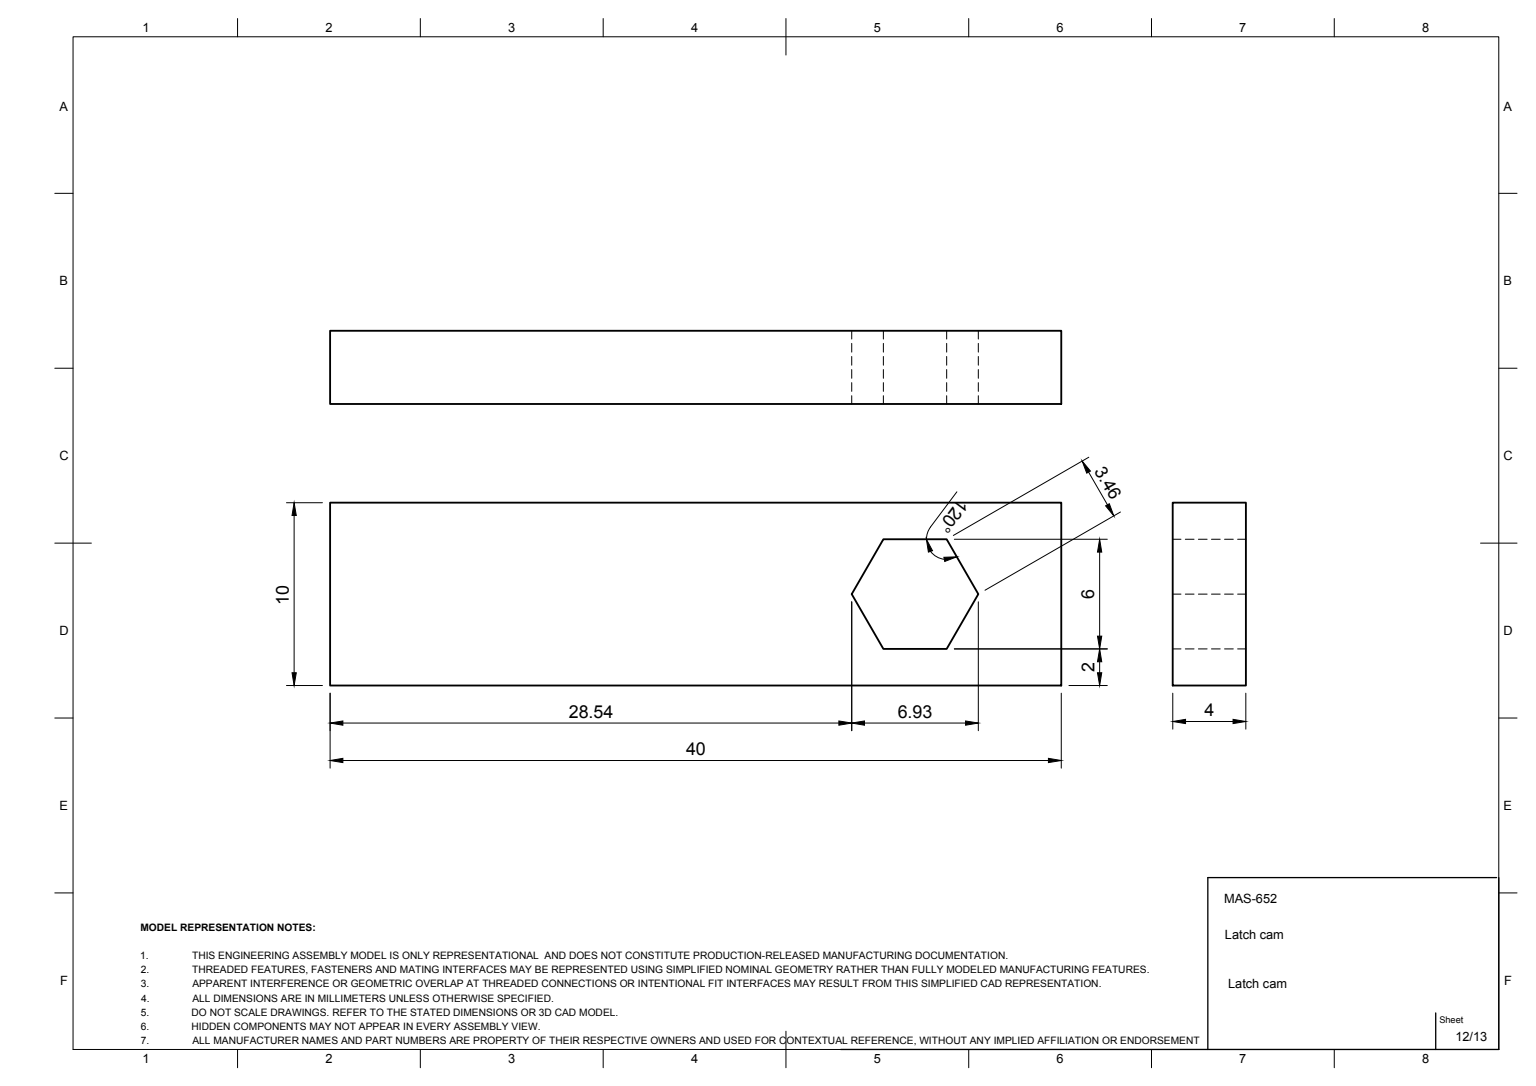
ISO-10303-21;
HEADER;
/* Generated by software containing ST-Developer
 * from STEP Tools, Inc. (www.steptools.com) 
 */

FILE_DESCRIPTION(
/* description */ ('Independent hinged machine back cover with retained hinge pins, perim
eter gasket and quarter-turn cam latch. Nominal cover 360 x 260 x 3 mm
, frame 430 x 300 x 20 mm. No guarding, structural or ingress rating a
ssigned.'),
/* implementation_level */ '2;1');

FILE_NAME(
/* name */ 'Latch cam.step',
/* time_stamp */ '2026-11-09T19:36:59-08:00',
/* author */ (''),
/* organization */ (''),
/* preprocessor_version */ 'ST-DEVELOPER v20.2',
/* originating_system */ 'Autodesk Translation Framework v15.17.0.0',
/* authorisation */ '');

FILE_SCHEMA (('AUTOMOTIVE_DESIGN { 1 0 10303 214 3 1 1 }'));
ENDSEC;

DATA;
#10=MECHANICAL_DESIGN_GEOMETRIC_PRESENTATION_REPRESENTATION('',(#202),#32627);
#166=SHAPE_REPRESENTATION_RELATIONSHIP('SRR','None',#32712,#184);
#184=ADVANCED_BREP_SHAPE_REPRESENTATION('',(#220),#32613);
#202=STYLED_ITEM('',(#32811),#220);
#220=MANIFOLD_SOLID_BREP('Body1',#8679);
#258=FACE_BOUND('',#1211,.T.);
#259=FACE_BOUND('',#1213,.T.);
#364=PLANE('',#9184);
#365=PLANE('',#9185);
#366=PLANE('',#9186);
#367=PLANE('',#9187);
#368=PLANE('',#9188);
#369=PLANE('',#9189);
#370=PLANE('',#9190);
#371=PLANE('',#9191);
#372=PLANE('',#9192);
#373=PLANE('',#9193);
#374=PLANE('',#9194);
#375=PLANE('',#9195);
#701=FACE_OUTER_BOUND('',#1200,.T.);
#702=FACE_OUTER_BOUND('',#1201,.T.);
#703=FACE_OUTER_BOUND('',#1202,.T.);
#704=FACE_OUTER_BOUND('',#1203,.T.);
#705=FACE_OUTER_BOUND('',#1204,.T.);
#706=FACE_OUTER_BOUND('',#1205,.T.);
#707=FACE_OUTER_BOUND('',#1206,.T.);
#708=FACE_OUTER_BOUND('',#1207,.T.);
#709=FACE_OUTER_BOUND('',#1208,.T.);
#710=FACE_OUTER_BOUND('',#1209,.T.);
#711=FACE_OUTER_BOUND('',#1210,.T.);
#712=FACE_OUTER_BOUND('',#1212,.T.);
#1200=EDGE_LOOP('',(#6753,#6754,#6755,#6756));
#1201=EDGE_LOOP('',(#6757,#6758,#6759,#6760));
#1202=EDGE_LOOP('',(#6761,#6762,#6763,#6764));
#1203=EDGE_LOOP('',(#6765,#6766,#6767,#6768));
#1204=EDGE_LOOP('',(#6769,#6770,#6771,#6772));
#1205=EDGE_LOOP('',(#6773,#6774,#6775,#6776));
#1206=EDGE_LOOP('',(#6777,#6778,#6779,#6780));
#1207=EDGE_LOOP('',(#6781,#6782,#6783,#6784));
#1208=EDGE_LOOP('',(#6785,#6786,#6787,#6788));
#1209=EDGE_LOOP('',(#6789,#6790,#6791,#6792));
#1210=EDGE_LOOP('',(#6793,#6794,#6795,#6796));
#1211=EDGE_LOOP('',(#6797,#6798,#6799,#6800,#6801,#6802));
#1212=EDGE_LOOP('',(#6803,#6804,#6805,#6806));
#1213=EDGE_LOOP('',(#6807,#6808,#6809,#6810,#6811,#6812));
#2446=LINE('',#24206,#2992);
#2447=LINE('',#24208,#2993);
#2448=LINE('',#24210,#2994);
#2449=LINE('',#24211,#2995);
#2450=LINE('',#24214,#2996);
#2451=LINE('',#24216,#2997);
#2452=LINE('',#24217,#2998);
#2453=LINE('',#24220,#2999);
#2454=LINE('',#24222,#3000);
#2455=LINE('',#24223,#3001);
#2456=LINE('',#24226,#3002);
#2457=LINE('',#24228,#3003);
#2458=LINE('',#24229,#3004);
#2459=LINE('',#24232,#3005);
#2460=LINE('',#24234,#3006);
#2461=LINE('',#24235,#3007);
#2462=LINE('',#24237,#3008);
#2463=LINE('',#24238,#3009);
#2464=LINE('',#24242,#3010);
#2465=LINE('',#24244,#3011);
#2466=LINE('',#24246,#3012);
#2467=LINE('',#24247,#3013);
#2468=LINE('',#24250,#3014);
#2469=LINE('',#24252,#3015);
#2470=LINE('',#24253,#3016);
#2471=LINE('',#24256,#3017);
#2472=LINE('',#24258,#3018);
#2473=LINE('',#24259,#3019);
#2474=LINE('',#24261,#3020);
#2475=LINE('',#24262,#3021);
#2992=VECTOR('',#10386,10.);
#2993=VECTOR('',#10387,10.);
#2994=VECTOR('',#10388,10.);
#2995=VECTOR('',#10389,10.);
#2996=VECTOR('',#10392,10.);
#2997=VECTOR('',#10393,10.);
#2998=VECTOR('',#10394,10.);
#2999=VECTOR('',#10397,10.);
#3000=VECTOR('',#10398,10.);
#3001=VECTOR('',#10399,10.);
#3002=VECTOR('',#10402,10.);
#3003=VECTOR('',#10403,10.);
#3004=VECTOR('',#10404,10.);
#3005=VECTOR('',#10407,10.);
#3006=VECTOR('',#10408,10.);
#3007=VECTOR('',#10409,10.);
#3008=VECTOR('',#10412,10.);
#3009=VECTOR('',#10413,10.);
#3010=VECTOR('',#10416,10.);
#3011=VECTOR('',#10417,10.);
#3012=VECTOR('',#10418,10.);
#3013=VECTOR('',#10419,10.);
#3014=VECTOR('',#10422,10.);
#3015=VECTOR('',#10423,10.);
#3016=VECTOR('',#10424,10.);
#3017=VECTOR('',#10427,10.);
#3018=VECTOR('',#10428,10.);
#3019=VECTOR('',#10429,10.);
#3020=VECTOR('',#10432,10.);
#3021=VECTOR('',#10433,10.);
#3729=VERTEX_POINT('',#24204);
#3730=VERTEX_POINT('',#24205);
#3731=VERTEX_POINT('',#24207);
#3732=VERTEX_POINT('',#24209);
#3733=VERTEX_POINT('',#24213);
#3734=VERTEX_POINT('',#24215);
#3735=VERTEX_POINT('',#24219);
#3736=VERTEX_POINT('',#24221);
#3737=VERTEX_POINT('',#24225);
#3738=VERTEX_POINT('',#24227);
#3739=VERTEX_POINT('',#24231);
#3740=VERTEX_POINT('',#24233);
#3741=VERTEX_POINT('',#24240);
#3742=VERTEX_POINT('',#24241);
#3743=VERTEX_POINT('',#24243);
#3744=VERTEX_POINT('',#24245);
#3745=VERTEX_POINT('',#24249);
#3746=VERTEX_POINT('',#24251);
#3747=VERTEX_POINT('',#24255);
#3748=VERTEX_POINT('',#24257);
#4800=EDGE_CURVE('',#3729,#3730,#2446,.T.);
#4801=EDGE_CURVE('',#3729,#3731,#2447,.T.);
#4802=EDGE_CURVE('',#3732,#3731,#2448,.T.);
#4803=EDGE_CURVE('',#3730,#3732,#2449,.T.);
#4804=EDGE_CURVE('',#3733,#3729,#2450,.T.);
#4805=EDGE_CURVE('',#3733,#3734,#2451,.T.);
#4806=EDGE_CURVE('',#3731,#3734,#2452,.T.);
#4807=EDGE_CURVE('',#3735,#3733,#2453,.T.);
#4808=EDGE_CURVE('',#3735,#3736,#2454,.T.);
#4809=EDGE_CURVE('',#3734,#3736,#2455,.T.);
#4810=EDGE_CURVE('',#3737,#3735,#2456,.T.);
#4811=EDGE_CURVE('',#3737,#3738,#2457,.T.);
#4812=EDGE_CURVE('',#3736,#3738,#2458,.T.);
#4813=EDGE_CURVE('',#3739,#3737,#2459,.T.);
#4814=EDGE_CURVE('',#3739,#3740,#2460,.T.);
#4815=EDGE_CURVE('',#3738,#3740,#2461,.T.);
#4816=EDGE_CURVE('',#3730,#3739,#2462,.T.);
#4817=EDGE_CURVE('',#3740,#3732,#2463,.T.);
#4818=EDGE_CURVE('',#3741,#3742,#2464,.T.);
#4819=EDGE_CURVE('',#3742,#3743,#2465,.T.);
#4820=EDGE_CURVE('',#3744,#3743,#2466,.T.);
#4821=EDGE_CURVE('',#3741,#3744,#2467,.T.);
#4822=EDGE_CURVE('',#3745,#3741,#2468,.T.);
#4823=EDGE_CURVE('',#3746,#3744,#2469,.T.);
#4824=EDGE_CURVE('',#3745,#3746,#2470,.T.);
#4825=EDGE_CURVE('',#3747,#3745,#2471,.T.);
#4826=EDGE_CURVE('',#3748,#3746,#2472,.T.);
#4827=EDGE_CURVE('',#3747,#3748,#2473,.T.);
#4828=EDGE_CURVE('',#3742,#3747,#2474,.T.);
#4829=EDGE_CURVE('',#3743,#3748,#2475,.T.);
#6753=ORIENTED_EDGE('',*,*,#4800,.F.);
#6754=ORIENTED_EDGE('',*,*,#4801,.T.);
#6755=ORIENTED_EDGE('',*,*,#4802,.F.);
#6756=ORIENTED_EDGE('',*,*,#4803,.F.);
#6757=ORIENTED_EDGE('',*,*,#4804,.F.);
#6758=ORIENTED_EDGE('',*,*,#4805,.T.);
#6759=ORIENTED_EDGE('',*,*,#4806,.F.);
#6760=ORIENTED_EDGE('',*,*,#4801,.F.);
#6761=ORIENTED_EDGE('',*,*,#4807,.F.);
#6762=ORIENTED_EDGE('',*,*,#4808,.T.);
#6763=ORIENTED_EDGE('',*,*,#4809,.F.);
#6764=ORIENTED_EDGE('',*,*,#4805,.F.);
#6765=ORIENTED_EDGE('',*,*,#4810,.F.);
#6766=ORIENTED_EDGE('',*,*,#4811,.T.);
#6767=ORIENTED_EDGE('',*,*,#4812,.F.);
#6768=ORIENTED_EDGE('',*,*,#4808,.F.);
#6769=ORIENTED_EDGE('',*,*,#4813,.F.);
#6770=ORIENTED_EDGE('',*,*,#4814,.T.);
#6771=ORIENTED_EDGE('',*,*,#4815,.F.);
#6772=ORIENTED_EDGE('',*,*,#4811,.F.);
#6773=ORIENTED_EDGE('',*,*,#4816,.F.);
#6774=ORIENTED_EDGE('',*,*,#4803,.T.);
#6775=ORIENTED_EDGE('',*,*,#4817,.F.);
#6776=ORIENTED_EDGE('',*,*,#4814,.F.);
#6777=ORIENTED_EDGE('',*,*,#4818,.T.);
#6778=ORIENTED_EDGE('',*,*,#4819,.T.);
#6779=ORIENTED_EDGE('',*,*,#4820,.F.);
#6780=ORIENTED_EDGE('',*,*,#4821,.F.);
#6781=ORIENTED_EDGE('',*,*,#4822,.T.);
#6782=ORIENTED_EDGE('',*,*,#4821,.T.);
#6783=ORIENTED_EDGE('',*,*,#4823,.F.);
#6784=ORIENTED_EDGE('',*,*,#4824,.F.);
#6785=ORIENTED_EDGE('',*,*,#4825,.T.);
#6786=ORIENTED_EDGE('',*,*,#4824,.T.);
#6787=ORIENTED_EDGE('',*,*,#4826,.F.);
#6788=ORIENTED_EDGE('',*,*,#4827,.F.);
#6789=ORIENTED_EDGE('',*,*,#4828,.T.);
#6790=ORIENTED_EDGE('',*,*,#4827,.T.);
#6791=ORIENTED_EDGE('',*,*,#4829,.F.);
#6792=ORIENTED_EDGE('',*,*,#4819,.F.);
#6793=ORIENTED_EDGE('',*,*,#4829,.T.);
#6794=ORIENTED_EDGE('',*,*,#4826,.T.);
#6795=ORIENTED_EDGE('',*,*,#4823,.T.);
#6796=ORIENTED_EDGE('',*,*,#4820,.T.);
#6797=ORIENTED_EDGE('',*,*,#4800,.T.);
#6798=ORIENTED_EDGE('',*,*,#4816,.T.);
#6799=ORIENTED_EDGE('',*,*,#4813,.T.);
#6800=ORIENTED_EDGE('',*,*,#4810,.T.);
#6801=ORIENTED_EDGE('',*,*,#4807,.T.);
#6802=ORIENTED_EDGE('',*,*,#4804,.T.);
#6803=ORIENTED_EDGE('',*,*,#4828,.F.);
#6804=ORIENTED_EDGE('',*,*,#4818,.F.);
#6805=ORIENTED_EDGE('',*,*,#4822,.F.);
#6806=ORIENTED_EDGE('',*,*,#4825,.F.);
#6807=ORIENTED_EDGE('',*,*,#4802,.T.);
#6808=ORIENTED_EDGE('',*,*,#4806,.T.);
#6809=ORIENTED_EDGE('',*,*,#4809,.T.);
#6810=ORIENTED_EDGE('',*,*,#4812,.T.);
#6811=ORIENTED_EDGE('',*,*,#4815,.T.);
#6812=ORIENTED_EDGE('',*,*,#4817,.T.);
#8449=ADVANCED_FACE('',(#701),#364,.F.);
#8450=ADVANCED_FACE('',(#702),#365,.F.);
#8451=ADVANCED_FACE('',(#703),#366,.F.);
#8452=ADVANCED_FACE('',(#704),#367,.F.);
#8453=ADVANCED_FACE('',(#705),#368,.F.);
#8454=ADVANCED_FACE('',(#706),#369,.F.);
#8455=ADVANCED_FACE('',(#707),#370,.T.);
#8456=ADVANCED_FACE('',(#708),#371,.T.);
#8457=ADVANCED_FACE('',(#709),#372,.T.);
#8458=ADVANCED_FACE('',(#710),#373,.T.);
#8459=ADVANCED_FACE('',(#711,#258),#374,.T.);
#8460=ADVANCED_FACE('',(#712,#259),#375,.F.);
#8679=CLOSED_SHELL('',(#8449,#8450,#8451,#8452,#8453,#8454,#8455,#8456,
#8457,#8458,#8459,#8460));
#9183=AXIS2_PLACEMENT_3D('',#24202,#10382,#10383);
#9184=AXIS2_PLACEMENT_3D('',#24203,#10384,#10385);
#9185=AXIS2_PLACEMENT_3D('',#24212,#10390,#10391);
#9186=AXIS2_PLACEMENT_3D('',#24218,#10395,#10396);
#9187=AXIS2_PLACEMENT_3D('',#24224,#10400,#10401);
#9188=AXIS2_PLACEMENT_3D('',#24230,#10405,#10406);
#9189=AXIS2_PLACEMENT_3D('',#24236,#10410,#10411);
#9190=AXIS2_PLACEMENT_3D('',#24239,#10414,#10415);
#9191=AXIS2_PLACEMENT_3D('',#24248,#10420,#10421);
#9192=AXIS2_PLACEMENT_3D('',#24254,#10425,#10426);
#9193=AXIS2_PLACEMENT_3D('',#24260,#10430,#10431);
#9194=AXIS2_PLACEMENT_3D('',#24263,#10434,#10435);
#9195=AXIS2_PLACEMENT_3D('',#24264,#10436,#10437);
#10382=DIRECTION('axis',(0.,0.,1.));
#10383=DIRECTION('refdir',(1.,0.,0.));
#10384=DIRECTION('center_axis',(0.866025403784439,0.5,0.));
#10385=DIRECTION('ref_axis',(0.5,-0.866025403784439,0.));
#10386=DIRECTION('',(0.5,-0.866025403784439,0.));
#10387=DIRECTION('',(0.,0.,-1.));
#10388=DIRECTION('',(-0.5,0.866025403784439,0.));
#10389=DIRECTION('',(0.,0.,-1.));
#10390=DIRECTION('center_axis',(1.60246890531964E-16,1.,0.));
#10391=DIRECTION('ref_axis',(1.,-1.60246890531964E-16,0.));
#10392=DIRECTION('',(1.,-1.60246890531964E-16,0.));
#10393=DIRECTION('',(0.,0.,-1.));
#10394=DIRECTION('',(-1.,1.60246890531964E-16,0.));
#10395=DIRECTION('center_axis',(-0.866025403784439,0.5,0.));
#10396=DIRECTION('ref_axis',(0.5,0.866025403784439,0.));
#10397=DIRECTION('',(0.5,0.866025403784439,0.));
#10398=DIRECTION('',(0.,0.,-1.));
#10399=DIRECTION('',(-0.5,-0.866025403784439,0.));
#10400=DIRECTION('center_axis',(-0.866025403784439,-0.5,0.));
#10401=DIRECTION('ref_axis',(-0.5,0.866025403784439,0.));
#10402=DIRECTION('',(-0.5,0.866025403784439,0.));
#10403=DIRECTION('',(0.,0.,-1.));
#10404=DIRECTION('',(0.5,-0.866025403784439,0.));
#10405=DIRECTION('center_axis',(-1.60246890531964E-16,-1.,0.));
#10406=DIRECTION('ref_axis',(-1.,1.60246890531964E-16,0.));
#10407=DIRECTION('',(-1.,1.60246890531964E-16,0.));
#10408=DIRECTION('',(0.,0.,-1.));
#10409=DIRECTION('',(1.,-1.60246890531964E-16,0.));
#10410=DIRECTION('center_axis',(0.866025403784439,-0.5,0.));
#10411=DIRECTION('ref_axis',(-0.5,-0.866025403784439,0.));
#10412=DIRECTION('',(-0.5,-0.866025403784439,0.));
#10413=DIRECTION('',(0.5,0.866025403784439,0.));
#10414=DIRECTION('center_axis',(0.,1.,0.));
#10415=DIRECTION('ref_axis',(-1.,0.,0.));
#10416=DIRECTION('',(-1.,0.,0.));
#10417=DIRECTION('',(0.,0.,1.));
#10418=DIRECTION('',(-1.,0.,0.));
#10419=DIRECTION('',(0.,0.,1.));
#10420=DIRECTION('center_axis',(1.,0.,0.));
#10421=DIRECTION('ref_axis',(0.,1.,0.));
#10422=DIRECTION('',(0.,1.,0.));
#10423=DIRECTION('',(0.,1.,0.));
#10424=DIRECTION('',(0.,0.,1.));
#10425=DIRECTION('center_axis',(0.,-1.,0.));
#10426=DIRECTION('ref_axis',(1.,0.,0.));
#10427=DIRECTION('',(1.,0.,0.));
#10428=DIRECTION('',(1.,0.,0.));
#10429=DIRECTION('',(0.,0.,1.));
#10430=DIRECTION('center_axis',(-1.,0.,0.));
#10431=DIRECTION('ref_axis',(0.,-1.,0.));
#10432=DIRECTION('',(0.,-1.,0.));
#10433=DIRECTION('',(0.,-1.,0.));
#10434=DIRECTION('center_axis',(0.,0.,1.));
#10435=DIRECTION('ref_axis',(1.,0.,0.));
#10436=DIRECTION('center_axis',(0.,0.,1.));
#10437=DIRECTION('ref_axis',(1.,0.,0.));
#24202=CARTESIAN_POINT('',(0.,0.,0.));
#24203=CARTESIAN_POINT('Origin',(1.73205080756888,3.,4.));
#24204=CARTESIAN_POINT('',(1.73205080756888,3.,4.));
#24205=CARTESIAN_POINT('',(3.46410161513775,0.,4.));
#24206=CARTESIAN_POINT('',(3.6650635094611,-0.348076211353315,4.));
#24207=CARTESIAN_POINT('',(1.73205080756888,3.,0.));
#24208=CARTESIAN_POINT('',(1.73205080756888,3.,4.));
#24209=CARTESIAN_POINT('',(3.46410161513775,0.,0.));
#24210=CARTESIAN_POINT('',(3.6650635094611,-0.348076211353316,0.));
#24211=CARTESIAN_POINT('',(3.46410161513775,0.,4.));
#24212=CARTESIAN_POINT('Origin',(-1.73205080756888,3.,4.));
#24213=CARTESIAN_POINT('',(-1.73205080756888,3.,4.));
#24214=CARTESIAN_POINT('',(5.13397459621556,3.,4.));
#24215=CARTESIAN_POINT('',(-1.73205080756888,3.,0.));
#24216=CARTESIAN_POINT('',(-1.73205080756888,3.,4.));
#24217=CARTESIAN_POINT('',(5.13397459621556,3.,0.));
#24218=CARTESIAN_POINT('Origin',(-3.46410161513775,5.55111512312578E-16,
4.));
#24219=CARTESIAN_POINT('',(-3.46410161513775,4.24230095489963E-16,4.));
#24220=CARTESIAN_POINT('',(-1.53108891324553,3.34807621135332,4.));
#24221=CARTESIAN_POINT('',(-3.46410161513775,5.55111512312578E-16,0.));
#24222=CARTESIAN_POINT('',(-3.46410161513775,4.24230095489963E-16,4.));
#24223=CARTESIAN_POINT('',(-1.53108891324553,3.34807621135332,-2.77555756156289E-16));
#24224=CARTESIAN_POINT('Origin',(-1.73205080756888,-3.,4.));
#24225=CARTESIAN_POINT('',(-1.73205080756888,-3.,4.));
#24226=CARTESIAN_POINT('',(-0.665063509461101,-4.84807621135331,4.));
#24227=CARTESIAN_POINT('',(-1.73205080756888,-3.,0.));
#24228=CARTESIAN_POINT('',(-1.73205080756888,-3.,4.));
#24229=CARTESIAN_POINT('',(-0.665063509461101,-4.84807621135332,-2.77555756156289E-16));
#24230=CARTESIAN_POINT('Origin',(1.73205080756888,-3.,4.));
#24231=CARTESIAN_POINT('',(1.73205080756888,-3.,4.));
#24232=CARTESIAN_POINT('',(6.86602540378444,-3.,4.));
#24233=CARTESIAN_POINT('',(1.73205080756888,-3.,0.));
#24234=CARTESIAN_POINT('',(1.73205080756888,-3.,4.));
#24235=CARTESIAN_POINT('',(6.86602540378444,-3.,0.));
#24236=CARTESIAN_POINT('Origin',(3.46410161513775,0.,4.));
#24237=CARTESIAN_POINT('',(4.53108891324554,1.84807621135332,4.));
#24238=CARTESIAN_POINT('',(4.53108891324553,1.84807621135332,0.));
#24239=CARTESIAN_POINT('Origin',(32.,5.,0.));
#24240=CARTESIAN_POINT('',(32.,5.,0.));
#24241=CARTESIAN_POINT('',(-8.,5.,0.));
#24242=CARTESIAN_POINT('',(32.,5.,0.));
#24243=CARTESIAN_POINT('',(-8.,5.,4.));
#24244=CARTESIAN_POINT('',(-8.,5.,0.));
#24245=CARTESIAN_POINT('',(32.,5.,4.));
#24246=CARTESIAN_POINT('',(32.,5.,4.));
#24247=CARTESIAN_POINT('',(32.,5.,0.));
#24248=CARTESIAN_POINT('Origin',(32.,-5.,0.));
#24249=CARTESIAN_POINT('',(32.,-5.,0.));
#24250=CARTESIAN_POINT('',(32.,-5.,0.));
#24251=CARTESIAN_POINT('',(32.,-5.,4.));
#24252=CARTESIAN_POINT('',(32.,-5.,4.));
#24253=CARTESIAN_POINT('',(32.,-5.,0.));
#24254=CARTESIAN_POINT('Origin',(-8.,-5.,0.));
#24255=CARTESIAN_POINT('',(-8.,-5.,0.));
#24256=CARTESIAN_POINT('',(-8.,-5.,0.));
#24257=CARTESIAN_POINT('',(-8.,-5.,4.));
#24258=CARTESIAN_POINT('',(-8.,-5.,4.));
#24259=CARTESIAN_POINT('',(-8.,-5.,0.));
#24260=CARTESIAN_POINT('Origin',(-8.,5.,0.));
#24261=CARTESIAN_POINT('',(-8.,5.,0.));
#24262=CARTESIAN_POINT('',(-8.,5.,4.));
#24263=CARTESIAN_POINT('Origin',(12.,0.,4.));
#24264=CARTESIAN_POINT('Origin',(12.,0.,0.));
#32593=UNCERTAINTY_MEASURE_WITH_UNIT(LENGTH_MEASURE(0.01),#32628,
'DISTANCE_ACCURACY_VALUE',
'Maximum model space distance between geometric entities at asserted c
onnectivities');
#32607=UNCERTAINTY_MEASURE_WITH_UNIT(LENGTH_MEASURE(0.01),#32628,
'DISTANCE_ACCURACY_VALUE',
'Maximum model space distance between geometric entities at asserted c
onnectivities');
#32613=(
GEOMETRIC_REPRESENTATION_CONTEXT(3)
GLOBAL_UNCERTAINTY_ASSIGNED_CONTEXT((#32593))
GLOBAL_UNIT_ASSIGNED_CONTEXT((#32628,#32630,#32631))
REPRESENTATION_CONTEXT('','3D')
);
#32627=(
GEOMETRIC_REPRESENTATION_CONTEXT(3)
GLOBAL_UNCERTAINTY_ASSIGNED_CONTEXT((#32607))
GLOBAL_UNIT_ASSIGNED_CONTEXT((#32628,#32630,#32631))
REPRESENTATION_CONTEXT('','3D')
);
#32628=(
LENGTH_UNIT()
NAMED_UNIT(*)
SI_UNIT(.MILLI.,.METRE.)
);
#32630=(
NAMED_UNIT(*)
PLANE_ANGLE_UNIT()
SI_UNIT($,.RADIAN.)
);
#32631=(
NAMED_UNIT(*)
SI_UNIT($,.STERADIAN.)
SOLID_ANGLE_UNIT()
);
#32637=SHAPE_DEFINITION_REPRESENTATION(#32656,#32712);
#32656=PRODUCT_DEFINITION_SHAPE('',$,#32732);
#32712=SHAPE_REPRESENTATION('',(#9183),#32613);
#32726=PRODUCT_DEFINITION_CONTEXT('part definition',#32785,'design');
#32732=PRODUCT_DEFINITION('Latch cam','Latch cam',#32751,#32726);
#32751=PRODUCT_DEFINITION_FORMATION('',$,#32792);
#32785=APPLICATION_CONTEXT(
'Core Data for Automotive Mechanical Design Process');
#32786=PRODUCT_CONTEXT('part definition',#32785,'mechanical');
#32792=PRODUCT('Latch cam','Latch cam',$,(#32786));
#32811=PRESENTATION_STYLE_ASSIGNMENT((#32818));
#32818=SURFACE_STYLE_USAGE(.BOTH.,#32825);
#32825=SURFACE_SIDE_STYLE('',(#32832));
#32832=SURFACE_STYLE_FILL_AREA(#32839);
#32839=FILL_AREA_STYLE('Sky blue',(#32846));
#32846=FILL_AREA_STYLE_COLOUR('Sky blue',#32853);
#32853=COLOUR_RGB('Sky blue',0.317647058823529,0.686274509803922,0.890196078431372);
ENDSEC;
END-ISO-10303-21;
